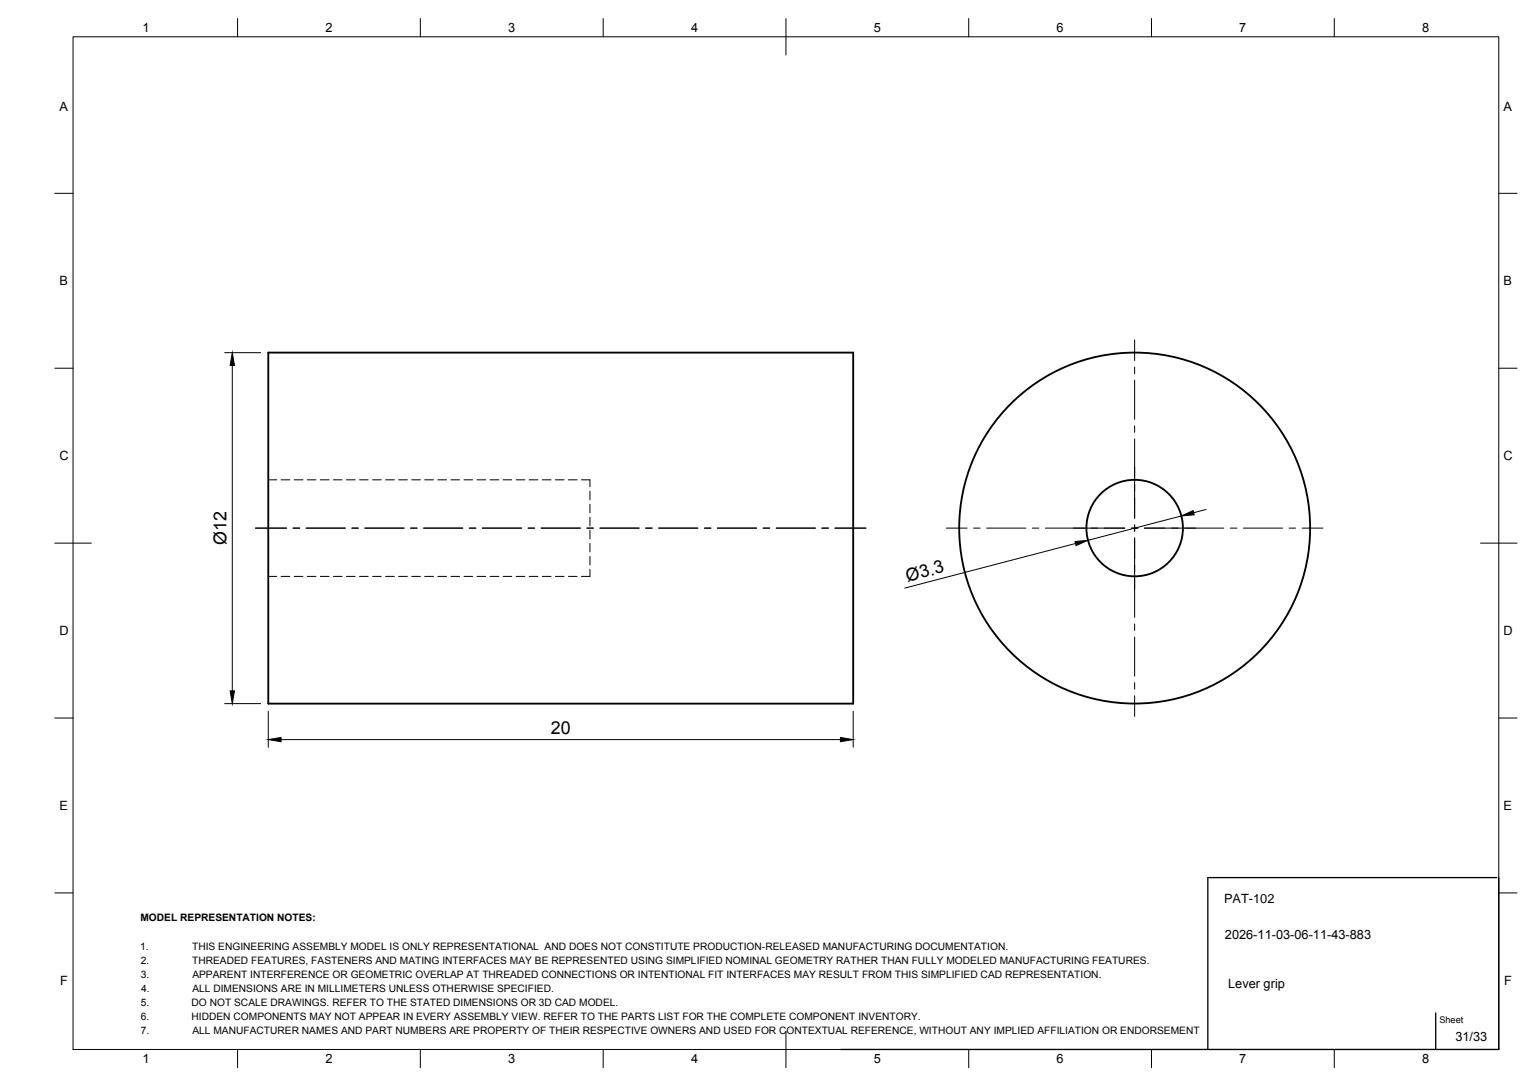
ISO-10303-21;
HEADER;
/* Generated by software containing ST-Developer
 * from STEP Tools, Inc. (www.steptools.com) 
 */

FILE_DESCRIPTION(
/* description */ ('Swing-away clamp arm'),
/* implementation_level */ '2;1');

FILE_NAME(
/* name */ 'Lever grip.step',
/* time_stamp */ '2026-10-28T03:26:03-07:00',
/* author */ (''),
/* organization */ (''),
/* preprocessor_version */ 'ST-DEVELOPER v20.2',
/* originating_system */ 'Autodesk Translation Framework v15.17.0.0',
/* authorisation */ '');

FILE_SCHEMA (('AUTOMOTIVE_DESIGN { 1 0 10303 214 3 1 1 }'));
ENDSEC;

DATA;
#10=MECHANICAL_DESIGN_GEOMETRIC_PRESENTATION_REPRESENTATION('',(#322),#10627);
#262=SHAPE_REPRESENTATION_RELATIONSHIP('SRR','None',#10763,#288);
#288=ADVANCED_BREP_SHAPE_REPRESENTATION('',(#355),#10622);
#322=STYLED_ITEM('',(#10972),#355);
#355=MANIFOLD_SOLID_BREP('Body1',#4929);
#451=FACE_BOUND('',#1302,.T.);
#608=PLANE('',#5768);
#609=PLANE('',#5772);
#610=PLANE('',#5773);
#898=FACE_OUTER_BOUND('',#1298,.T.);
#899=FACE_OUTER_BOUND('',#1299,.T.);
#900=FACE_OUTER_BOUND('',#1300,.T.);
#901=FACE_OUTER_BOUND('',#1301,.T.);
#902=FACE_OUTER_BOUND('',#1303,.T.);
#1298=EDGE_LOOP('',(#4337,#4338,#4339,#4340));
#1299=EDGE_LOOP('',(#4341));
#1300=EDGE_LOOP('',(#4342,#4343,#4344,#4345));
#1301=EDGE_LOOP('',(#4346));
#1302=EDGE_LOOP('',(#4347));
#1303=EDGE_LOOP('',(#4348));
#1620=LINE('',#10359,#1942);
#1621=LINE('',#10366,#1943);
#1942=VECTOR('',#7227,0.164999999999999);
#1943=VECTOR('',#7236,0.6);
#2235=CIRCLE('',#5766,0.164999999999999);
#2236=CIRCLE('',#5767,0.164999999999999);
#2237=CIRCLE('',#5770,0.6);
#2238=CIRCLE('',#5771,0.6);
#2622=VERTEX_POINT('',#10356);
#2623=VERTEX_POINT('',#10358);
#2624=VERTEX_POINT('',#10363);
#2625=VERTEX_POINT('',#10365);
#3201=EDGE_CURVE('',#2622,#2622,#2235,.T.);
#3202=EDGE_CURVE('',#2622,#2623,#1620,.T.);
#3203=EDGE_CURVE('',#2623,#2623,#2236,.T.);
#3204=EDGE_CURVE('',#2624,#2624,#2237,.T.);
#3205=EDGE_CURVE('',#2624,#2625,#1621,.T.);
#3206=EDGE_CURVE('',#2625,#2625,#2238,.T.);
#4337=ORIENTED_EDGE('',*,*,#3201,.F.);
#4338=ORIENTED_EDGE('',*,*,#3202,.T.);
#4339=ORIENTED_EDGE('',*,*,#3203,.F.);
#4340=ORIENTED_EDGE('',*,*,#3202,.F.);
#4341=ORIENTED_EDGE('',*,*,#3201,.T.);
#4342=ORIENTED_EDGE('',*,*,#3204,.F.);
#4343=ORIENTED_EDGE('',*,*,#3205,.T.);
#4344=ORIENTED_EDGE('',*,*,#3206,.T.);
#4345=ORIENTED_EDGE('',*,*,#3205,.F.);
#4346=ORIENTED_EDGE('',*,*,#3204,.T.);
#4347=ORIENTED_EDGE('',*,*,#3203,.T.);
#4348=ORIENTED_EDGE('',*,*,#3206,.F.);
#4582=CYLINDRICAL_SURFACE('',#5765,0.164999999999999);
#4583=CYLINDRICAL_SURFACE('',#5769,0.6);
#4853=ADVANCED_FACE('',(#898),#4582,.F.);
#4854=ADVANCED_FACE('',(#899),#608,.T.);
#4855=ADVANCED_FACE('',(#900),#4583,.T.);
#4856=ADVANCED_FACE('',(#901,#451),#609,.T.);
#4857=ADVANCED_FACE('',(#902),#610,.F.);
#4929=CLOSED_SHELL('',(#4853,#4854,#4855,#4856,#4857));
#5764=AXIS2_PLACEMENT_3D('',#10354,#7221,#7222);
#5765=AXIS2_PLACEMENT_3D('',#10355,#7223,#7224);
#5766=AXIS2_PLACEMENT_3D('',#10357,#7225,#7226);
#5767=AXIS2_PLACEMENT_3D('',#10360,#7228,#7229);
#5768=AXIS2_PLACEMENT_3D('',#10361,#7230,#7231);
#5769=AXIS2_PLACEMENT_3D('',#10362,#7232,#7233);
#5770=AXIS2_PLACEMENT_3D('',#10364,#7234,#7235);
#5771=AXIS2_PLACEMENT_3D('',#10367,#7237,#7238);
#5772=AXIS2_PLACEMENT_3D('',#10368,#7239,#7240);
#5773=AXIS2_PLACEMENT_3D('',#10369,#7241,#7242);
#7221=DIRECTION('axis',(0.,0.,1.));
#7222=DIRECTION('refdir',(1.,0.,0.));
#7223=DIRECTION('center_axis',(0.,1.,0.));
#7224=DIRECTION('ref_axis',(1.,0.,0.));
#7225=DIRECTION('center_axis',(0.,1.,0.));
#7226=DIRECTION('ref_axis',(1.,0.,0.));
#7227=DIRECTION('',(0.,1.,0.));
#7228=DIRECTION('center_axis',(0.,-1.,0.));
#7229=DIRECTION('ref_axis',(1.,0.,0.));
#7230=DIRECTION('center_axis',(0.,1.,0.));
#7231=DIRECTION('ref_axis',(1.,0.,0.));
#7232=DIRECTION('center_axis',(0.,1.,0.));
#7233=DIRECTION('ref_axis',(1.,0.,0.));
#7234=DIRECTION('center_axis',(0.,1.,0.));
#7235=DIRECTION('ref_axis',(1.,0.,0.));
#7236=DIRECTION('',(0.,-1.,0.));
#7237=DIRECTION('center_axis',(0.,1.,0.));
#7238=DIRECTION('ref_axis',(1.,0.,0.));
#7239=DIRECTION('center_axis',(0.,1.,0.));
#7240=DIRECTION('ref_axis',(1.,0.,0.));
#7241=DIRECTION('center_axis',(0.,1.,0.));
#7242=DIRECTION('ref_axis',(1.,0.,0.));
#10354=CARTESIAN_POINT('',(0.,0.,0.));
#10355=CARTESIAN_POINT('Origin',(8.5,-3.3,10.5));
#10356=CARTESIAN_POINT('',(8.335,-3.3,10.5));
#10357=CARTESIAN_POINT('Origin',(8.5,-3.3,10.5));
#10358=CARTESIAN_POINT('',(8.335,-2.2,10.5));
#10359=CARTESIAN_POINT('',(8.335,-3.3,10.5));
#10360=CARTESIAN_POINT('Origin',(8.5,-2.2,10.5));
#10361=CARTESIAN_POINT('Origin',(8.5,-3.3,10.5));
#10362=CARTESIAN_POINT('Origin',(8.5,-4.2,10.5));
#10363=CARTESIAN_POINT('',(7.9,-2.2,10.5));
#10364=CARTESIAN_POINT('Origin',(8.5,-2.2,10.5));
#10365=CARTESIAN_POINT('',(7.9,-4.2,10.5));
#10366=CARTESIAN_POINT('',(7.9,-4.2,10.5));
#10367=CARTESIAN_POINT('Origin',(8.5,-4.2,10.5));
#10368=CARTESIAN_POINT('Origin',(8.5,-2.2,10.5));
#10369=CARTESIAN_POINT('Origin',(8.5,-4.2,10.5));
#10590=UNCERTAINTY_MEASURE_WITH_UNIT(LENGTH_MEASURE(0.001),#10628,
'DISTANCE_ACCURACY_VALUE',
'Maximum model space distance between geometric entities at asserted c
onnectivities');
#10595=UNCERTAINTY_MEASURE_WITH_UNIT(LENGTH_MEASURE(0.001),#10628,
'DISTANCE_ACCURACY_VALUE',
'Maximum model space distance between geometric entities at asserted c
onnectivities');
#10622=(
GEOMETRIC_REPRESENTATION_CONTEXT(3)
GLOBAL_UNCERTAINTY_ASSIGNED_CONTEXT((#10590))
GLOBAL_UNIT_ASSIGNED_CONTEXT((#10628,#10630,#10631))
REPRESENTATION_CONTEXT('','3D')
);
#10627=(
GEOMETRIC_REPRESENTATION_CONTEXT(3)
GLOBAL_UNCERTAINTY_ASSIGNED_CONTEXT((#10595))
GLOBAL_UNIT_ASSIGNED_CONTEXT((#10628,#10630,#10631))
REPRESENTATION_CONTEXT('','3D')
);
#10628=(
LENGTH_UNIT()
NAMED_UNIT(*)
SI_UNIT(.CENTI.,.METRE.)
);
#10630=(
NAMED_UNIT(*)
PLANE_ANGLE_UNIT()
SI_UNIT($,.RADIAN.)
);
#10631=(
NAMED_UNIT(*)
SI_UNIT($,.STERADIAN.)
SOLID_ANGLE_UNIT()
);
#10658=SHAPE_DEFINITION_REPRESENTATION(#10704,#10763);
#10704=PRODUCT_DEFINITION_SHAPE('',$,#10795);
#10763=SHAPE_REPRESENTATION('',(#5764),#10622);
#10768=PRODUCT_DEFINITION_CONTEXT('part definition',#10863,'design');
#10795=PRODUCT_DEFINITION('Lever grip','Lever grip',#10826,#10768);
#10826=PRODUCT_DEFINITION_FORMATION('',$,#10891);
#10863=APPLICATION_CONTEXT(
'Core Data for Automotive Mechanical Design Process');
#10864=PRODUCT_CONTEXT('part definition',#10863,'mechanical');
#10891=PRODUCT('Lever grip','Lever grip','Lever grip',(#10864));
#10966=COLOUR_RGB('Black',0.12,0.14,0.17);
#10967=FILL_AREA_STYLE_COLOUR('',#10966);
#10968=FILL_AREA_STYLE('',(#10967));
#10969=SURFACE_STYLE_FILL_AREA(#10968);
#10970=SURFACE_SIDE_STYLE('',(#10969));
#10971=SURFACE_STYLE_USAGE(.BOTH.,#10970);
#10972=PRESENTATION_STYLE_ASSIGNMENT((#10971));
ENDSEC;
END-ISO-10303-21;
